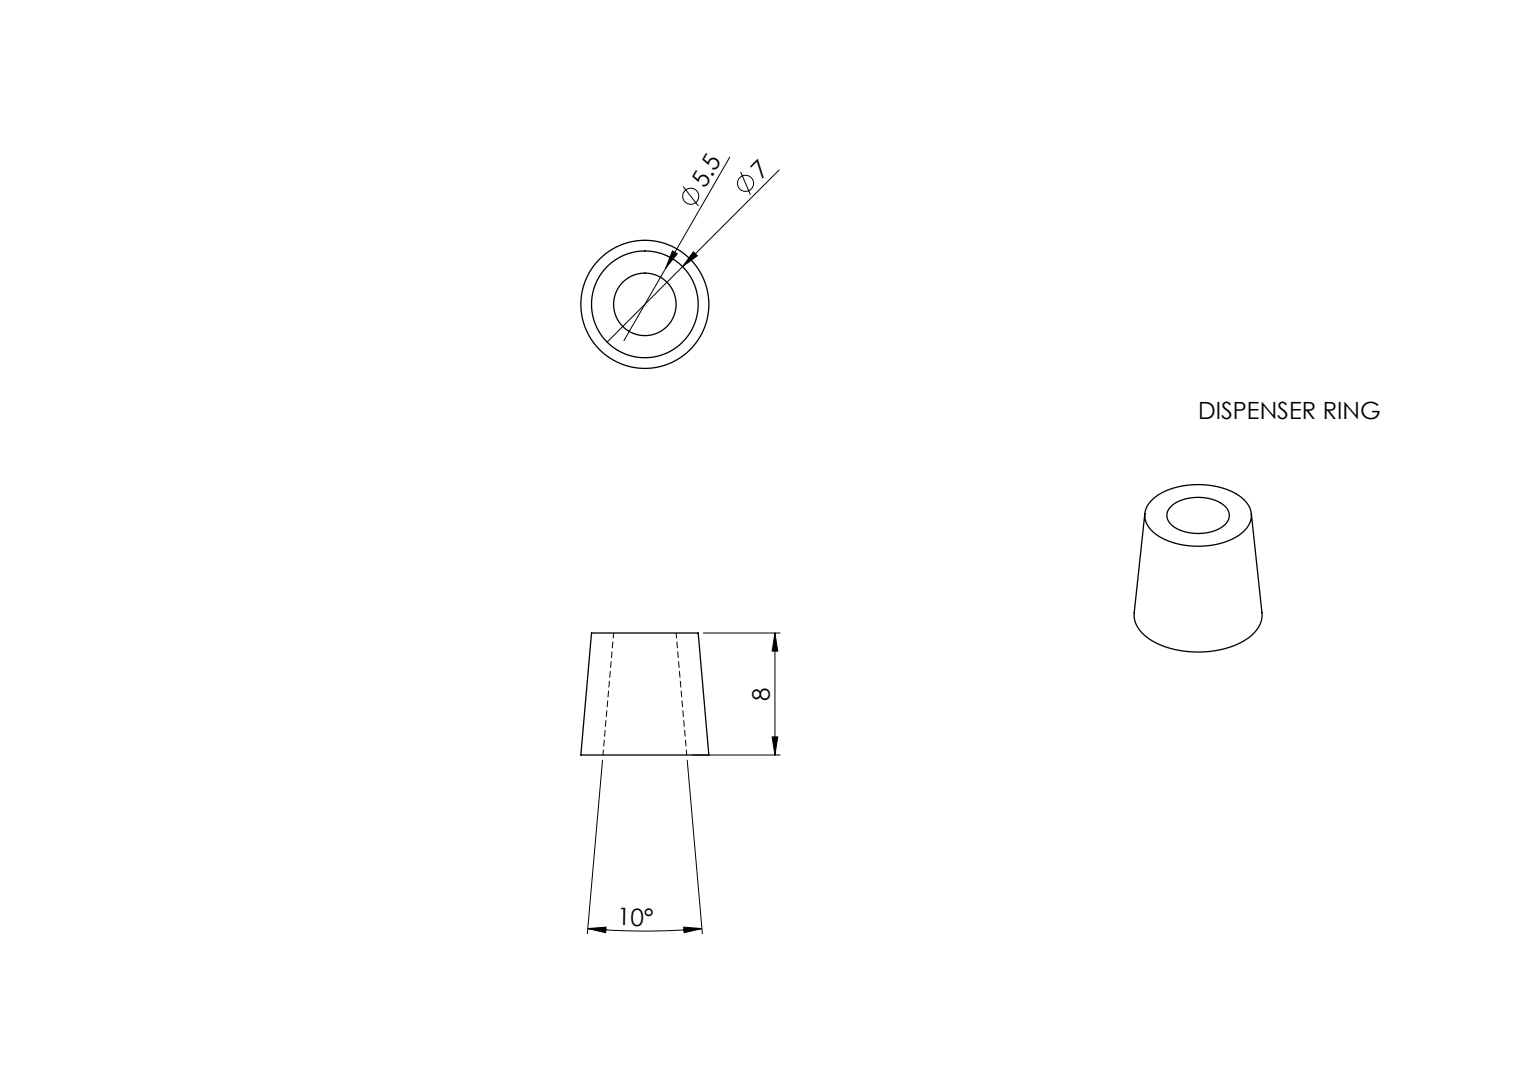
ISO-10303-21;
HEADER;
FILE_DESCRIPTION (('STEP AP214'),
    '1' );
FILE_NAME ('dispenser ring.step',
    '2026-10-27T10:49:47',
    ( '' ),
    ( '' ),
    'SwSTEP 2.0',
    'SolidWorks 2026',
    '' );
FILE_SCHEMA (( 'AUTOMOTIVE_DESIGN' ));
ENDSEC;

DATA;
#207=AXIS2_PLACEMENT_3D ( 'NONE', #5032, #1556, #5225 ) ;
#220=PRODUCT_DEFINITION_CONTEXT ( 'detailed design', #4323, 'design' ) ;
#232=ORIENTED_EDGE ( 'NONE', *, *, #8410, .T. ) ;
#303=FACE_BOUND ( 'NONE', #8931, .T. ) ;
#450=VECTOR ( 'NONE', #5852, 1000.000000000000000 ) ;
#565=PRODUCT_DEFINITION_FORMATION_WITH_SPECIFIED_SOURCE ( 'ANY', '', #2108, .NOT_KNOWN. ) ;
#578=ADVANCED_FACE ( 'NONE', ( #8381, #5440 ), #8422, .T. ) ;
#590=ORIENTED_EDGE ( 'NONE', *, *, #1735, .F. ) ;
#606=DIRECTION ( 'NONE',  ( 0.000000000000000000, -1.000000000000000000, 0.000000000000000000 ) ) ;
#704=CARTESIAN_POINT ( 'NONE',  ( 0.000000000000000000, -28.00000000000000000, -2.750000000000000000 ) ) ;
#734=DIRECTION ( 'NONE',  ( 1.067350013832299517E-17, -0.9961946980917455452, 0.08715574274765836016 ) ) ;
#747=AXIS2_PLACEMENT_3D ( 'NONE', #6440, #4909, #7757 ) ;
#769=EDGE_LOOP ( 'NONE', ( #7449, #1488, #232, #2395 ) ) ;
#867=EDGE_CURVE ( 'NONE', #8201, #5024, #2277, .T. ) ;
#888=AXIS2_PLACEMENT_3D ( 'NONE', #4026, #9081, #6861 ) ;
#919=CARTESIAN_POINT ( 'NONE',  ( 3.367778697655221012E-16, -28.00000000000000000, 2.750000000000000000 ) ) ;
#933=EDGE_CURVE ( 'NONE', #2936, #3199, #6596, .T. ) ;
#955=DIRECTION ( 'NONE',  ( 0.000000000000000000, -1.000000000000000000, 0.000000000000000000 ) ) ;
#987=DIRECTION ( 'NONE',  ( 0.000000000000000000, -1.000000000000000000, 0.000000000000000000 ) ) ;
#1057=AXIS2_PLACEMENT_3D ( 'NONE', #2801, #6450, #3581 ) ;
#1218=FACE_OUTER_BOUND ( 'NONE', #1222, .T. ) ;
#1222=EDGE_LOOP ( 'NONE', ( #5319, #5073, #7446, #1505 ) ) ;
#1266=ORIENTED_EDGE ( 'NONE', *, *, #4371, .F. ) ;
#1290=ADVANCED_FACE ( 'NONE', ( #2880 ), #5743, .F. ) ;
#1303=DIRECTION ( 'NONE',  ( 0.000000000000000000, 0.000000000000000000, -1.000000000000000000 ) ) ;
#1403=EDGE_CURVE ( 'NONE', #6870, #7184, #6991, .T. ) ;
#1488=ORIENTED_EDGE ( 'NONE', *, *, #2428, .F. ) ;
#1505=ORIENTED_EDGE ( 'NONE', *, *, #8954, .F. ) ;
#1556=DIRECTION ( 'NONE',  ( 0.000000000000000000, -1.000000000000000000, 0.000000000000000000 ) ) ;
#1614=UNCERTAINTY_MEASURE_WITH_UNIT (LENGTH_MEASURE( 1.000000000000000082E-05 ), #8120, 'distance_accuracy_value', 'NONE');
#1657=DIRECTION ( 'NONE',  ( 0.000000000000000000, -0.000000000000000000, -1.000000000000000000 ) ) ;
#1678=CIRCLE ( 'NONE', #5541, 2.750000000000000000 ) ;
#1683=AXIS2_PLACEMENT_3D ( 'NONE', #7363, #987, #4483 ) ;
#1704=VERTEX_POINT ( 'NONE', #7451 ) ;
#1735=EDGE_CURVE ( 'NONE', #3199, #5007, #9069, .T. ) ;
#1745=( GEOMETRIC_REPRESENTATION_CONTEXT ( 3 ) GLOBAL_UNCERTAINTY_ASSIGNED_CONTEXT ( ( #5793 ) ) GLOBAL_UNIT_ASSIGNED_CONTEXT ( ( #3922, #7355, #8883 ) ) REPRESENTATION_CONTEXT ( 'NONE', 'WORKASPACE' ) );
#1781=( LENGTH_UNIT ( ) NAMED_UNIT ( * ) SI_UNIT ( .MILLI., .METRE. ) );
#1805=ADVANCED_FACE ( 'NONE', ( #1218 ), #5208, .T. ) ;
#1959=PRODUCT_CONTEXT ( 'NONE', #8129, 'mechanical' ) ;
#2027=CARTESIAN_POINT ( 'NONE',  ( 0.000000000000000000, -28.00000000000000000, 0.000000000000000000 ) ) ;
#2050=CARTESIAN_POINT ( 'NONE',  ( 0.000000000000000000, -28.00000000000000000, 0.000000000000000000 ) ) ;
#2108=PRODUCT ( 'dispenser ring', 'dispenser ring', '', ( #1959 ) ) ;
#2134=ADVANCED_FACE ( 'NONE', ( #3493 ), #5635, .F. ) ;
#2259=( NAMED_UNIT ( * ) SI_UNIT ( $, .STERADIAN. ) SOLID_ANGLE_UNIT ( ) );
#2261=PLANE ( 'NONE',  #7002 ) ;
#2264=UNCERTAINTY_MEASURE_WITH_UNIT (LENGTH_MEASURE( 1.000000000000000082E-05 ), #1781, 'distance_accuracy_value', 'NONE');
#2277=CIRCLE ( 'NONE', #2586, 4.199909308207394609 ) ;
#2340=STYLED_ITEM ( 'NONE', ( #3137 ), #4954 ) ;
#2351=DIRECTION ( 'NONE',  ( 0.000000000000000000, -1.000000000000000000, 0.000000000000000000 ) ) ;
#2367=DIRECTION ( 'NONE',  ( 1.067350013832299517E-17, -0.9961946980917455452, 0.08715574274765836016 ) ) ;
#2395=ORIENTED_EDGE ( 'NONE', *, *, #4371, .T. ) ;
#2420=CARTESIAN_POINT ( 'NONE',  ( 0.000000000000000000, -20.00000000000000000, -3.500000000000000444 ) ) ;
#2428=EDGE_CURVE ( 'NONE', #1704, #2936, #3714, .T. ) ;
#2478=FILL_AREA_STYLE ('',( #3045 ) ) ;
#2561=ADVANCED_FACE ( 'NONE', ( #303, #5931 ), #2261, .F. ) ;
#2586=AXIS2_PLACEMENT_3D ( 'NONE', #5804, #5243, #5941 ) ;
#2604=CONICAL_SURFACE ( 'NONE', #207, 3.500000000000000444, 0.08726646259971666819 ) ;
#2754=CARTESIAN_POINT ( 'NONE',  ( 4.714834644010547828E-16, -20.00000000000000000, 3.500000000000000444 ) ) ;
#2759=DIRECTION ( 'NONE',  ( 0.000000000000000000, -1.000000000000000000, 0.000000000000000000 ) ) ;
#2761=ORIENTED_EDGE ( 'NONE', *, *, #8274, .T. ) ;
#2787=EDGE_LOOP ( 'NONE', ( #1266, #590 ) ) ;
#2801=CARTESIAN_POINT ( 'NONE',  ( 0.000000000000000000, -28.00000000000000000, 0.000000000000000000 ) ) ;
#2812=AXIS2_PLACEMENT_3D ( 'NONE', #2836, #8503, #4950 ) ;
#2836=CARTESIAN_POINT ( 'NONE',  ( 0.000000000000000000, -28.00000000000000000, 0.000000000000000000 ) ) ;
#2868=CARTESIAN_POINT ( 'NONE',  ( 2.939207850660410271E-16, -20.00000000000000000, 2.050090691792606279 ) ) ;
#2880=FACE_OUTER_BOUND ( 'NONE', #8908, .T. ) ;
#2934=CARTESIAN_POINT ( 'NONE',  ( 4.286263797015737088E-16, -20.00000000000000000, 3.500000000000000444 ) ) ;
#2936=VERTEX_POINT ( 'NONE', #2868 ) ;
#2965=AXIS2_PLACEMENT_3D ( 'NONE', #8720, #2351, #5181 ) ;
#3045=FILL_AREA_STYLE_COLOUR ( '', #6641 ) ;
#3119=CIRCLE ( 'NONE', #4298, 3.500000000000000444 ) ;
#3127=EDGE_LOOP ( 'NONE', ( #3914, #7118 ) ) ;
#3137=PRESENTATION_STYLE_ASSIGNMENT (( #7260 ) ) ;
#3199=VERTEX_POINT ( 'NONE', #8713 ) ;
#3213=ORIENTED_EDGE ( 'NONE', *, *, #8410, .F. ) ;
#3337=LINE ( 'NONE', #6211, #5187 ) ;
#3419=STYLED_ITEM('',(#9218),#8209);
#3475=ORIENTED_EDGE ( 'NONE', *, *, #5195, .T. ) ;
#3493=FACE_OUTER_BOUND ( 'NONE', #769, .T. ) ;
#3505=EDGE_CURVE ( 'NONE', #7184, #8201, #7816, .T. ) ;
#3581=DIRECTION ( 'NONE',  ( 0.000000000000000000, 0.000000000000000000, -1.000000000000000000 ) ) ;
#3704=MECHANICAL_DESIGN_GEOMETRIC_PRESENTATION_REPRESENTATION('',(#3419),#8602);
#3714=CIRCLE ( 'NONE', #7274, 2.050090691792606279 ) ;
#3815=ORIENTED_EDGE ( 'NONE', *, *, #2428, .T. ) ;
#3852=EDGE_LOOP ( 'NONE', ( #7270, #6818, #5417, #3946 ) ) ;
#3914=ORIENTED_EDGE ( 'NONE', *, *, #1403, .F. ) ;
#3922=( LENGTH_UNIT ( ) NAMED_UNIT ( * ) SI_UNIT ( .MILLI., .METRE. ) );
#3946=ORIENTED_EDGE ( 'NONE', *, *, #867, .F. ) ;
#4011=CARTESIAN_POINT ( 'NONE',  ( 0.000000000000000000, -28.00000000000000000, 0.000000000000000000 ) ) ;
#4026=CARTESIAN_POINT ( 'NONE',  ( 0.000000000000000000, 0.000000000000000000, 0.000000000000000000 ) ) ;
#4176=AXIS2_PLACEMENT_3D ( 'NONE', #4011, #7498, #5441 ) ;
#4298=AXIS2_PLACEMENT_3D ( 'NONE', #8181, #6074, #8911 ) ;
#4323=APPLICATION_CONTEXT ( 'automotive_design' ) ;
#4331=PRODUCT_DEFINITION ( 'UNKNOWN', '', #565, #220 ) ;
#4371=EDGE_CURVE ( 'NONE', #5007, #3199, #1678, .T. ) ;
#4384=SHAPE_REPRESENTATION ( 'dispenser ring', ( #888 ), #1745 ) ;
#4474=SURFACE_STYLE_FILL_AREA ( #2478 ) ;
#4483=DIRECTION ( 'NONE',  ( 0.000000000000000000, 0.000000000000000000, -1.000000000000000000 ) ) ;
#4570=ORIENTED_EDGE ( 'NONE', *, *, #933, .T. ) ;
#4611=ORIENTED_EDGE ( 'NONE', *, *, #867, .T. ) ;
#4673=ORIENTED_EDGE ( 'NONE', *, *, #1735, .T. ) ;
#4717=( GEOMETRIC_REPRESENTATION_CONTEXT ( 3 ) GLOBAL_UNCERTAINTY_ASSIGNED_CONTEXT ( ( #2264 ) ) GLOBAL_UNIT_ASSIGNED_CONTEXT ( ( #1781, #5958, #7311 ) ) REPRESENTATION_CONTEXT ( 'NONE', 'WORKASPACE' ) );
#4862=DIRECTION ( 'NONE',  ( 0.000000000000000000, 0.000000000000000000, -1.000000000000000000 ) ) ;
#4901=ORIENTED_EDGE ( 'NONE', *, *, #8274, .F. ) ;
#4909=DIRECTION ( 'NONE',  ( 0.000000000000000000, -1.000000000000000000, 0.000000000000000000 ) ) ;
#4950=DIRECTION ( 'NONE',  ( 0.000000000000000000, 0.000000000000000000, -1.000000000000000000 ) ) ;
#4954=ADVANCED_BREP_SHAPE_REPRESENTATION ( '', ( #8209, #888 ), #1745 ) ;
#5007=VERTEX_POINT ( 'NONE', #704 ) ;
#5019=CARTESIAN_POINT ( 'NONE',  ( 0.000000000000000000, -28.00000000000000000, -4.199909308207393721 ) ) ;
#5024=VERTEX_POINT ( 'NONE', #5019 ) ;
#5032=CARTESIAN_POINT ( 'NONE',  ( 0.000000000000000000, -20.00000000000000000, 0.000000000000000000 ) ) ;
#5073=ORIENTED_EDGE ( 'NONE', *, *, #3505, .T. ) ;
#5080=FACE_OUTER_BOUND ( 'NONE', #3852, .T. ) ;
#5085=CARTESIAN_POINT ( 'NONE',  ( 5.143405491005359555E-16, -28.00000000000000000, 4.199909308207393721 ) ) ;
#5089=VECTOR ( 'NONE', #2367, 1000.000000000000000 ) ;
#5102=CARTESIAN_POINT ( 'NONE',  ( 0.000000000000000000, -20.00000000000000000, -3.500000000000000444 ) ) ;
#5181=DIRECTION ( 'NONE',  ( 0.000000000000000000, 0.000000000000000000, -1.000000000000000000 ) ) ;
#5187=VECTOR ( 'NONE', #5367, 1000.000000000000000 ) ;
#5195=EDGE_CURVE ( 'NONE', #5024, #8201, #7326, .T. ) ;
#5208=CONICAL_SURFACE ( 'NONE', #7288, 3.500000000000000444, 0.08726646259971666819 ) ;
#5225=DIRECTION ( 'NONE',  ( 0.000000000000000000, 0.000000000000000000, -1.000000000000000000 ) ) ;
#5243=DIRECTION ( 'NONE',  ( 0.000000000000000000, -1.000000000000000000, 0.000000000000000000 ) ) ;
#5319=ORIENTED_EDGE ( 'NONE', *, *, #1403, .T. ) ;
#5329=PRODUCT_DEFINITION_SHAPE ( 'NONE', 'NONE',  #4331 ) ;
#5367=DIRECTION ( 'NONE',  ( 0.000000000000000000, -0.9961946980917455452, -0.08715574274765836016 ) ) ;
#5385=SHAPE_DEFINITION_REPRESENTATION ( #5329, #4384 ) ;
#5417=ORIENTED_EDGE ( 'NONE', *, *, #8954, .T. ) ;
#5440=FACE_OUTER_BOUND ( 'NONE', #5781, .T. ) ;
#5441=DIRECTION ( 'NONE',  ( 0.000000000000000000, 0.000000000000000000, -1.000000000000000000 ) ) ;
#5494=CLOSED_SHELL ( 'NONE', ( #1290, #1805, #6438, #578, #2561, #2134 ) ) ;
#5541=AXIS2_PLACEMENT_3D ( 'NONE', #2027, #6255, #7042 ) ;
#5602=MECHANICAL_DESIGN_GEOMETRIC_PRESENTATION_REPRESENTATION('',(#2340),#4717);
#5609=DIRECTION ( 'NONE',  ( 0.000000000000000000, -1.000000000000000000, 0.000000000000000000 ) ) ;
#5635=CONICAL_SURFACE ( 'NONE', #1057, 2.750000000000000000, 0.08726646259971666819 ) ;
#5743=CONICAL_SURFACE ( 'NONE', #2812, 2.750000000000000000, 0.08726646259971666819 ) ;
#5781=EDGE_LOOP ( 'NONE', ( #3475, #4611 ) ) ;
#5793=UNCERTAINTY_MEASURE_WITH_UNIT (LENGTH_MEASURE( 1.000000000000000082E-05 ), #3922, 'distance_accuracy_value', 'NONE');
#5804=CARTESIAN_POINT ( 'NONE',  ( 0.000000000000000000, -28.00000000000000000, 0.000000000000000000 ) ) ;
#5852=DIRECTION ( 'NONE',  ( 0.000000000000000000, -0.9961946980917455452, -0.08715574274765836016 ) ) ;
#5931=FACE_OUTER_BOUND ( 'NONE', #3127, .T. ) ;
#5941=DIRECTION ( 'NONE',  ( 0.000000000000000000, 0.000000000000000000, -1.000000000000000000 ) ) ;
#5945=LINE ( 'NONE', #5102, #450 ) ;
#5958=( NAMED_UNIT ( * ) PLANE_ANGLE_UNIT ( ) SI_UNIT ( $, .RADIAN. ) );
#6074=DIRECTION ( 'NONE',  ( 0.000000000000000000, -1.000000000000000000, 0.000000000000000000 ) ) ;
#6211=CARTESIAN_POINT ( 'NONE',  ( 0.000000000000000000, -28.00000000000000000, -2.750000000000000000 ) ) ;
#6255=DIRECTION ( 'NONE',  ( 0.000000000000000000, -1.000000000000000000, 0.000000000000000000 ) ) ;
#6287=AXIS2_PLACEMENT_3D ( 'NONE', #2050, #606, #8335 ) ;
#6438=ADVANCED_FACE ( 'NONE', ( #5080 ), #2604, .T. ) ;
#6440=CARTESIAN_POINT ( 'NONE',  ( 0.000000000000000000, -20.00000000000000000, 0.000000000000000000 ) ) ;
#6450=DIRECTION ( 'NONE',  ( -0.000000000000000000, -1.000000000000000000, -0.000000000000000000 ) ) ;
#6560=SURFACE_SIDE_STYLE ('',( #4474 ) ) ;
#6596=LINE ( 'NONE', #919, #5089 ) ;
#6641=COLOUR_RGB ( '',0.8941176470588234615, 0.8941176470588234615, 0.8941176470588234615 ) ;
#6699=SHAPE_REPRESENTATION_RELATIONSHIP ( 'NONE' , 'NONE' ,  #4384, #4954 ) ;
#6818=ORIENTED_EDGE ( 'NONE', *, *, #7770, .T. ) ;
#6861=DIRECTION ( 'NONE',  ( 1.000000000000000000, 0.000000000000000000, 0.000000000000000000 ) ) ;
#6870=VERTEX_POINT ( 'NONE', #2420 ) ;
#6969=CIRCLE ( 'NONE', #2965, 2.050090691792606279 ) ;
#6991=CIRCLE ( 'NONE', #747, 3.500000000000000444 ) ;
#7002=AXIS2_PLACEMENT_3D ( 'NONE', #7329, #955, #1657 ) ;
#7042=DIRECTION ( 'NONE',  ( 0.000000000000000000, 0.000000000000000000, -1.000000000000000000 ) ) ;
#7118=ORIENTED_EDGE ( 'NONE', *, *, #7770, .F. ) ;
#7184=VERTEX_POINT ( 'NONE', #2754 ) ;
#7260=SURFACE_STYLE_USAGE ( .BOTH. , #6560 ) ;
#7270=ORIENTED_EDGE ( 'NONE', *, *, #3505, .F. ) ;
#7274=AXIS2_PLACEMENT_3D ( 'NONE', #7710, #5609, #4862 ) ;
#7288=AXIS2_PLACEMENT_3D ( 'NONE', #7593, #2759, #1303 ) ;
#7311=( NAMED_UNIT ( * ) SI_UNIT ( $, .STERADIAN. ) SOLID_ANGLE_UNIT ( ) );
#7326=CIRCLE ( 'NONE', #1683, 4.199909308207394609 ) ;
#7329=CARTESIAN_POINT ( 'NONE',  ( 0.000000000000000000, -20.00000000000000000, 0.000000000000000000 ) ) ;
#7355=( NAMED_UNIT ( * ) PLANE_ANGLE_UNIT ( ) SI_UNIT ( $, .RADIAN. ) );
#7363=CARTESIAN_POINT ( 'NONE',  ( 0.000000000000000000, -28.00000000000000000, 0.000000000000000000 ) ) ;
#7446=ORIENTED_EDGE ( 'NONE', *, *, #5195, .F. ) ;
#7449=ORIENTED_EDGE ( 'NONE', *, *, #933, .F. ) ;
#7451=CARTESIAN_POINT ( 'NONE',  ( 0.000000000000000000, -20.00000000000000000, -2.050090691792606279 ) ) ;
#7498=DIRECTION ( 'NONE',  ( 0.000000000000000000, -1.000000000000000000, 0.000000000000000000 ) ) ;
#7593=CARTESIAN_POINT ( 'NONE',  ( 0.000000000000000000, -20.00000000000000000, 0.000000000000000000 ) ) ;
#7710=CARTESIAN_POINT ( 'NONE',  ( 0.000000000000000000, -20.00000000000000000, 0.000000000000000000 ) ) ;
#7757=DIRECTION ( 'NONE',  ( 0.000000000000000000, 0.000000000000000000, -1.000000000000000000 ) ) ;
#7770=EDGE_CURVE ( 'NONE', #7184, #6870, #3119, .T. ) ;
#7816=LINE ( 'NONE', #2934, #8912 ) ;
#7977=( NAMED_UNIT ( * ) PLANE_ANGLE_UNIT ( ) SI_UNIT ( $, .RADIAN. ) );
#8120=( LENGTH_UNIT ( ) NAMED_UNIT ( * ) SI_UNIT ( .MILLI., .METRE. ) );
#8129=APPLICATION_CONTEXT ( 'automotive_design' ) ;
#8181=CARTESIAN_POINT ( 'NONE',  ( 0.000000000000000000, -20.00000000000000000, 0.000000000000000000 ) ) ;
#8201=VERTEX_POINT ( 'NONE', #5085 ) ;
#8209=MANIFOLD_SOLID_BREP ( 'Cut-Extrude1', #5494 ) ;
#8274=EDGE_CURVE ( 'NONE', #2936, #1704, #6969, .T. ) ;
#8335=DIRECTION ( 'NONE',  ( 0.000000000000000000, -0.000000000000000000, -1.000000000000000000 ) ) ;
#8381=FACE_BOUND ( 'NONE', #2787, .T. ) ;
#8410=EDGE_CURVE ( 'NONE', #1704, #5007, #3337, .T. ) ;
#8422=PLANE ( 'NONE',  #6287 ) ;
#8503=DIRECTION ( 'NONE',  ( -0.000000000000000000, -1.000000000000000000, -0.000000000000000000 ) ) ;
#8602=( GEOMETRIC_REPRESENTATION_CONTEXT ( 3 ) GLOBAL_UNCERTAINTY_ASSIGNED_CONTEXT ( ( #1614 ) ) GLOBAL_UNIT_ASSIGNED_CONTEXT ( ( #8120, #7977, #2259 ) ) REPRESENTATION_CONTEXT ( 'NONE', 'WORKASPACE' ) );
#8713=CARTESIAN_POINT ( 'NONE',  ( 3.367778697655221012E-16, -28.00000000000000000, 2.750000000000000000 ) ) ;
#8720=CARTESIAN_POINT ( 'NONE',  ( 0.000000000000000000, -20.00000000000000000, 0.000000000000000000 ) ) ;
#8883=( NAMED_UNIT ( * ) SI_UNIT ( $, .STERADIAN. ) SOLID_ANGLE_UNIT ( ) );
#8908=EDGE_LOOP ( 'NONE', ( #4901, #4570, #4673, #3213 ) ) ;
#8911=DIRECTION ( 'NONE',  ( 0.000000000000000000, 0.000000000000000000, -1.000000000000000000 ) ) ;
#8912=VECTOR ( 'NONE', #734, 1000.000000000000000 ) ;
#8931=EDGE_LOOP ( 'NONE', ( #3815, #2761 ) ) ;
#8954=EDGE_CURVE ( 'NONE', #6870, #5024, #5945, .T. ) ;
#9069=CIRCLE ( 'NONE', #4176, 2.750000000000000000 ) ;
#9081=DIRECTION ( 'NONE',  ( 0.000000000000000000, 0.000000000000000000, 1.000000000000000000 ) ) ;
#9212=COLOUR_RGB('Sky Blue',0.24,0.69,0.87);
#9213=FILL_AREA_STYLE_COLOUR('',#9212);
#9214=FILL_AREA_STYLE('',(#9213));
#9215=SURFACE_STYLE_FILL_AREA(#9214);
#9216=SURFACE_SIDE_STYLE('',(#9215));
#9217=SURFACE_STYLE_USAGE(.BOTH.,#9216);
#9218=PRESENTATION_STYLE_ASSIGNMENT((#9217));
ENDSEC;
END-ISO-10303-21;
